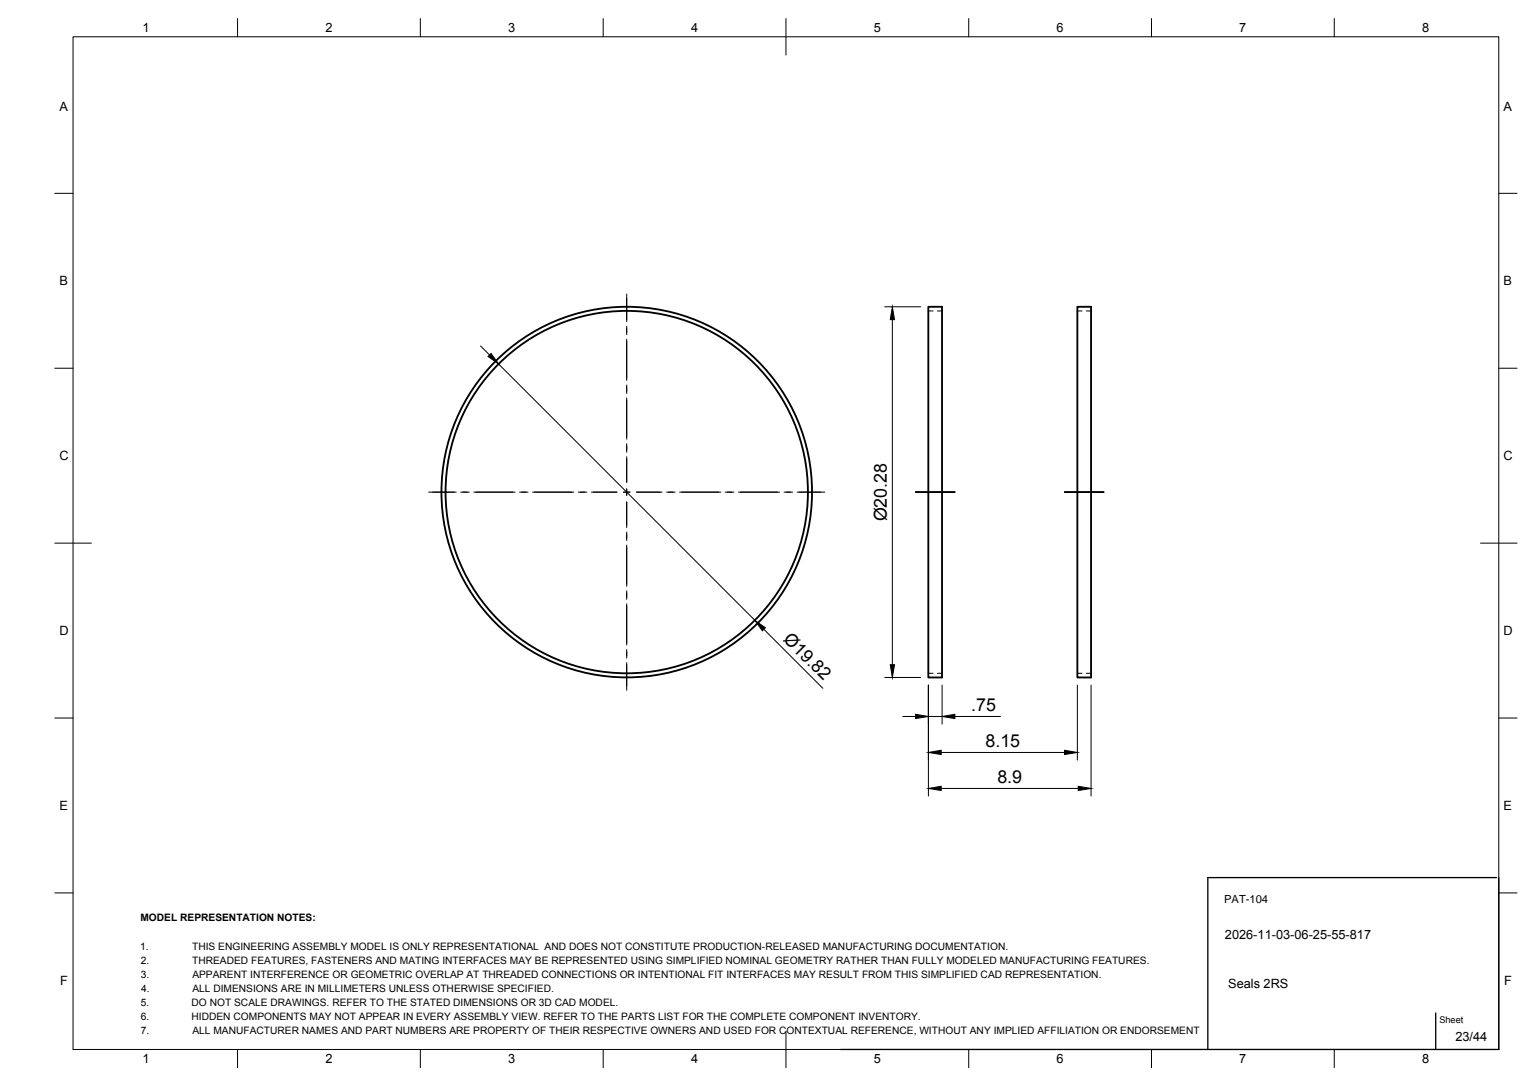
ISO-10303-21;
HEADER;
/* Generated by software containing ST-Developer
 * from STEP Tools, Inc. (www.steptools.com) 
 */

FILE_DESCRIPTION(
/* description */ ('Timing belt drive module 2 mm Pitch Timing 20T-40T'),

/* implementation_level */ '2;1');

FILE_NAME(
/* name */ 'Seals 2RS.step',
/* time_stamp */ '2026-10-28T03:25:12-07:00',
/* author */ (''),
/* organization */ (''),
/* preprocessor_version */ 'ST-DEVELOPER v20.2',
/* originating_system */ 'Autodesk Translation Framework v15.17.0.0',
/* authorisation */ '');

FILE_SCHEMA (('AUTOMOTIVE_DESIGN { 1 0 10303 214 3 1 1 }'));
ENDSEC;

DATA;
#10=MECHANICAL_DESIGN_GEOMETRIC_PRESENTATION_REPRESENTATION('',(#551,#552),#17830);
#458=SHAPE_REPRESENTATION_RELATIONSHIP('SRR','None',#18029,#501);
#501=ADVANCED_BREP_SHAPE_REPRESENTATION('',(#609,#610),#17804);
#551=STYLED_ITEM('',(#18317),#609);
#552=STYLED_ITEM('',(#18317),#610);
#609=MANIFOLD_SOLID_BREP('Body1',#9008);
#610=MANIFOLD_SOLID_BREP('Body2',#9009);
#714=FACE_BOUND('',#1770,.T.);
#715=FACE_BOUND('',#1773,.T.);
#716=FACE_BOUND('',#1776,.T.);
#717=FACE_BOUND('',#1779,.T.);
#866=PLANE('',#9989);
#867=PLANE('',#9994);
#868=PLANE('',#9997);
#869=PLANE('',#10002);
#1171=FACE_OUTER_BOUND('',#1769,.T.);
#1172=FACE_OUTER_BOUND('',#1771,.T.);
#1173=FACE_OUTER_BOUND('',#1772,.T.);
#1174=FACE_OUTER_BOUND('',#1774,.T.);
#1175=FACE_OUTER_BOUND('',#1775,.T.);
#1176=FACE_OUTER_BOUND('',#1777,.T.);
#1177=FACE_OUTER_BOUND('',#1778,.T.);
#1178=FACE_OUTER_BOUND('',#1780,.T.);
#1769=EDGE_LOOP('',(#6729));
#1770=EDGE_LOOP('',(#6730));
#1771=EDGE_LOOP('',(#6731,#6732,#6733,#6734));
#1772=EDGE_LOOP('',(#6735));
#1773=EDGE_LOOP('',(#6736));
#1774=EDGE_LOOP('',(#6737,#6738,#6739,#6740));
#1775=EDGE_LOOP('',(#6741));
#1776=EDGE_LOOP('',(#6742));
#1777=EDGE_LOOP('',(#6743,#6744,#6745,#6746));
#1778=EDGE_LOOP('',(#6747));
#1779=EDGE_LOOP('',(#6748));
#1780=EDGE_LOOP('',(#6749,#6750,#6751,#6752));
#2380=CIRCLE('',#9990,1.013815);
#2381=CIRCLE('',#9991,0.991185);
#2382=CIRCLE('',#9993,1.013815);
#2383=CIRCLE('',#9995,0.991185);
#2384=CIRCLE('',#9998,1.013815);
#2385=CIRCLE('',#9999,0.991185);
#2386=CIRCLE('',#10001,1.013815);
#2387=CIRCLE('',#10003,0.991185);
#3010=LINE('',#15258,#3488);
#3011=LINE('',#15263,#3489);
#3012=LINE('',#15272,#3490);
#3013=LINE('',#15277,#3491);
#3488=VECTOR('',#11985,1.013815);
#3489=VECTOR('',#11992,0.991185);
#3490=VECTOR('',#12003,1.013815);
#3491=VECTOR('',#12010,0.991185);
#4074=VERTEX_POINT('',#15251);
#4075=VERTEX_POINT('',#15253);
#4076=VERTEX_POINT('',#15256);
#4077=VERTEX_POINT('',#15260);
#4078=VERTEX_POINT('',#15265);
#4079=VERTEX_POINT('',#15267);
#4080=VERTEX_POINT('',#15270);
#4081=VERTEX_POINT('',#15274);
#5047=EDGE_CURVE('',#4074,#4074,#2380,.T.);
#5048=EDGE_CURVE('',#4075,#4075,#2381,.T.);
#5049=EDGE_CURVE('',#4076,#4076,#2382,.T.);
#5050=EDGE_CURVE('',#4076,#4074,#3010,.T.);
#5051=EDGE_CURVE('',#4077,#4077,#2383,.T.);
#5052=EDGE_CURVE('',#4077,#4075,#3011,.T.);
#5053=EDGE_CURVE('',#4078,#4078,#2384,.T.);
#5054=EDGE_CURVE('',#4079,#4079,#2385,.T.);
#5055=EDGE_CURVE('',#4080,#4080,#2386,.T.);
#5056=EDGE_CURVE('',#4080,#4078,#3012,.T.);
#5057=EDGE_CURVE('',#4081,#4081,#2387,.T.);
#5058=EDGE_CURVE('',#4081,#4079,#3013,.T.);
#6729=ORIENTED_EDGE('',*,*,#5047,.F.);
#6730=ORIENTED_EDGE('',*,*,#5048,.T.);
#6731=ORIENTED_EDGE('',*,*,#5049,.F.);
#6732=ORIENTED_EDGE('',*,*,#5050,.T.);
#6733=ORIENTED_EDGE('',*,*,#5047,.T.);
#6734=ORIENTED_EDGE('',*,*,#5050,.F.);
#6735=ORIENTED_EDGE('',*,*,#5049,.T.);
#6736=ORIENTED_EDGE('',*,*,#5051,.F.);
#6737=ORIENTED_EDGE('',*,*,#5051,.T.);
#6738=ORIENTED_EDGE('',*,*,#5052,.T.);
#6739=ORIENTED_EDGE('',*,*,#5048,.F.);
#6740=ORIENTED_EDGE('',*,*,#5052,.F.);
#6741=ORIENTED_EDGE('',*,*,#5053,.F.);
#6742=ORIENTED_EDGE('',*,*,#5054,.T.);
#6743=ORIENTED_EDGE('',*,*,#5055,.F.);
#6744=ORIENTED_EDGE('',*,*,#5056,.T.);
#6745=ORIENTED_EDGE('',*,*,#5053,.T.);
#6746=ORIENTED_EDGE('',*,*,#5056,.F.);
#6747=ORIENTED_EDGE('',*,*,#5055,.T.);
#6748=ORIENTED_EDGE('',*,*,#5057,.F.);
#6749=ORIENTED_EDGE('',*,*,#5057,.T.);
#6750=ORIENTED_EDGE('',*,*,#5058,.T.);
#6751=ORIENTED_EDGE('',*,*,#5054,.F.);
#6752=ORIENTED_EDGE('',*,*,#5058,.F.);
#8275=CYLINDRICAL_SURFACE('',#9992,1.013815);
#8276=CYLINDRICAL_SURFACE('',#9996,0.991185);
#8277=CYLINDRICAL_SURFACE('',#10000,1.013815);
#8278=CYLINDRICAL_SURFACE('',#10004,0.991185);
#8669=ADVANCED_FACE('',(#1171,#714),#866,.T.);
#8670=ADVANCED_FACE('',(#1172),#8275,.T.);
#8671=ADVANCED_FACE('',(#1173,#715),#867,.T.);
#8672=ADVANCED_FACE('',(#1174),#8276,.F.);
#8673=ADVANCED_FACE('',(#1175,#716),#868,.T.);
#8674=ADVANCED_FACE('',(#1176),#8277,.T.);
#8675=ADVANCED_FACE('',(#1177,#717),#869,.T.);
#8676=ADVANCED_FACE('',(#1178),#8278,.F.);
#9008=CLOSED_SHELL('',(#8669,#8670,#8671,#8672));
#9009=CLOSED_SHELL('',(#8673,#8674,#8675,#8676));
#9988=AXIS2_PLACEMENT_3D('',#15249,#11973,#11974);
#9989=AXIS2_PLACEMENT_3D('',#15250,#11975,#11976);
#9990=AXIS2_PLACEMENT_3D('',#15252,#11977,#11978);
#9991=AXIS2_PLACEMENT_3D('',#15254,#11979,#11980);
#9992=AXIS2_PLACEMENT_3D('',#15255,#11981,#11982);
#9993=AXIS2_PLACEMENT_3D('',#15257,#11983,#11984);
#9994=AXIS2_PLACEMENT_3D('',#15259,#11986,#11987);
#9995=AXIS2_PLACEMENT_3D('',#15261,#11988,#11989);
#9996=AXIS2_PLACEMENT_3D('',#15262,#11990,#11991);
#9997=AXIS2_PLACEMENT_3D('',#15264,#11993,#11994);
#9998=AXIS2_PLACEMENT_3D('',#15266,#11995,#11996);
#9999=AXIS2_PLACEMENT_3D('',#15268,#11997,#11998);
#10000=AXIS2_PLACEMENT_3D('',#15269,#11999,#12000);
#10001=AXIS2_PLACEMENT_3D('',#15271,#12001,#12002);
#10002=AXIS2_PLACEMENT_3D('',#15273,#12004,#12005);
#10003=AXIS2_PLACEMENT_3D('',#15275,#12006,#12007);
#10004=AXIS2_PLACEMENT_3D('',#15276,#12008,#12009);
#11973=DIRECTION('axis',(0.,0.,1.));
#11974=DIRECTION('refdir',(1.,0.,0.));
#11975=DIRECTION('center_axis',(0.,1.,0.));
#11976=DIRECTION('ref_axis',(0.,0.,1.));
#11977=DIRECTION('center_axis',(0.,-1.,0.));
#11978=DIRECTION('ref_axis',(1.,0.,0.));
#11979=DIRECTION('center_axis',(0.,-1.,0.));
#11980=DIRECTION('ref_axis',(1.,0.,0.));
#11981=DIRECTION('center_axis',(0.,-1.,0.));
#11982=DIRECTION('ref_axis',(1.,0.,0.));
#11983=DIRECTION('center_axis',(0.,-1.,0.));
#11984=DIRECTION('ref_axis',(1.,0.,0.));
#11985=DIRECTION('',(0.,1.,0.));
#11986=DIRECTION('center_axis',(0.,-1.,0.));
#11987=DIRECTION('ref_axis',(0.,0.,-1.));
#11988=DIRECTION('center_axis',(0.,-1.,0.));
#11989=DIRECTION('ref_axis',(1.,0.,0.));
#11990=DIRECTION('center_axis',(0.,-1.,0.));
#11991=DIRECTION('ref_axis',(1.,0.,0.));
#11992=DIRECTION('',(0.,1.,0.));
#11993=DIRECTION('center_axis',(0.,1.,0.));
#11994=DIRECTION('ref_axis',(0.,0.,1.));
#11995=DIRECTION('center_axis',(0.,-1.,0.));
#11996=DIRECTION('ref_axis',(1.,0.,0.));
#11997=DIRECTION('center_axis',(0.,-1.,0.));
#11998=DIRECTION('ref_axis',(1.,0.,0.));
#11999=DIRECTION('center_axis',(0.,-1.,0.));
#12000=DIRECTION('ref_axis',(1.,0.,0.));
#12001=DIRECTION('center_axis',(0.,-1.,0.));
#12002=DIRECTION('ref_axis',(1.,0.,0.));
#12003=DIRECTION('',(0.,1.,0.));
#12004=DIRECTION('center_axis',(0.,-1.,0.));
#12005=DIRECTION('ref_axis',(0.,0.,-1.));
#12006=DIRECTION('center_axis',(0.,-1.,0.));
#12007=DIRECTION('ref_axis',(1.,0.,0.));
#12008=DIRECTION('center_axis',(0.,-1.,0.));
#12009=DIRECTION('ref_axis',(1.,0.,0.));
#12010=DIRECTION('',(0.,1.,0.));
#15249=CARTESIAN_POINT('',(0.,0.,0.));
#15250=CARTESIAN_POINT('Origin',(1.013815,0.445,0.));
#15251=CARTESIAN_POINT('',(-1.013815,0.445,-1.24156529467757E-16));
#15252=CARTESIAN_POINT('Origin',(0.,0.445,0.));
#15253=CARTESIAN_POINT('',(-0.991185,0.445,-1.21385153761287E-16));
#15254=CARTESIAN_POINT('Origin',(0.,0.445,0.));
#15255=CARTESIAN_POINT('Origin',(0.,0.4075,0.));
#15256=CARTESIAN_POINT('',(-1.013815,0.37,-1.24156529467757E-16));
#15257=CARTESIAN_POINT('Origin',(0.,0.37,0.));
#15258=CARTESIAN_POINT('',(-1.013815,0.4075,-1.24156529467757E-16));
#15259=CARTESIAN_POINT('Origin',(0.991185,0.37,0.));
#15260=CARTESIAN_POINT('',(-0.991185,0.37,-1.21385153761287E-16));
#15261=CARTESIAN_POINT('Origin',(0.,0.37,0.));
#15262=CARTESIAN_POINT('Origin',(0.,0.4075,0.));
#15263=CARTESIAN_POINT('',(-0.991185,0.4075,-1.21385153761287E-16));
#15264=CARTESIAN_POINT('Origin',(1.013815,-0.37,0.));
#15265=CARTESIAN_POINT('',(-1.013815,-0.37,-1.24156529467757E-16));
#15266=CARTESIAN_POINT('Origin',(0.,-0.37,0.));
#15267=CARTESIAN_POINT('',(-0.991185,-0.37,-1.21385153761287E-16));
#15268=CARTESIAN_POINT('Origin',(0.,-0.37,0.));
#15269=CARTESIAN_POINT('Origin',(0.,-0.4075,0.));
#15270=CARTESIAN_POINT('',(-1.013815,-0.445,-1.24156529467757E-16));
#15271=CARTESIAN_POINT('Origin',(0.,-0.445,0.));
#15272=CARTESIAN_POINT('',(-1.013815,-0.4075,-1.24156529467757E-16));
#15273=CARTESIAN_POINT('Origin',(0.991185,-0.445,0.));
#15274=CARTESIAN_POINT('',(-0.991185,-0.445,-1.21385153761287E-16));
#15275=CARTESIAN_POINT('Origin',(0.,-0.445,0.));
#15276=CARTESIAN_POINT('Origin',(0.,-0.4075,0.));
#15277=CARTESIAN_POINT('',(-0.991185,-0.4075,-1.21385153761287E-16));
#17754=UNCERTAINTY_MEASURE_WITH_UNIT(LENGTH_MEASURE(0.001),#17831,
'DISTANCE_ACCURACY_VALUE',
'Maximum model space distance between geometric entities at asserted c
onnectivities');
#17780=UNCERTAINTY_MEASURE_WITH_UNIT(LENGTH_MEASURE(0.001),#17831,
'DISTANCE_ACCURACY_VALUE',
'Maximum model space distance between geometric entities at asserted c
onnectivities');
#17804=(
GEOMETRIC_REPRESENTATION_CONTEXT(3)
GLOBAL_UNCERTAINTY_ASSIGNED_CONTEXT((#17754))
GLOBAL_UNIT_ASSIGNED_CONTEXT((#17831,#17833,#17834))
REPRESENTATION_CONTEXT('','3D')
);
#17830=(
GEOMETRIC_REPRESENTATION_CONTEXT(3)
GLOBAL_UNCERTAINTY_ASSIGNED_CONTEXT((#17780))
GLOBAL_UNIT_ASSIGNED_CONTEXT((#17831,#17833,#17834))
REPRESENTATION_CONTEXT('','3D')
);
#17831=(
LENGTH_UNIT()
NAMED_UNIT(*)
SI_UNIT(.CENTI.,.METRE.)
);
#17833=(
NAMED_UNIT(*)
PLANE_ANGLE_UNIT()
SI_UNIT($,.RADIAN.)
);
#17834=(
NAMED_UNIT(*)
SI_UNIT($,.STERADIAN.)
SOLID_ANGLE_UNIT()
);
#17858=SHAPE_DEFINITION_REPRESENTATION(#17907,#18029);
#17907=PRODUCT_DEFINITION_SHAPE('',$,#18079);
#18029=SHAPE_REPRESENTATION('',(#9988),#17804);
#18055=PRODUCT_DEFINITION_CONTEXT('part definition',#18204,'design');
#18079=PRODUCT_DEFINITION('Seals 2RS','Seals 2RS',#18128,#18055);
#18128=PRODUCT_DEFINITION_FORMATION('',$,#18229);
#18204=APPLICATION_CONTEXT(
'Core Data for Automotive Mechanical Design Process');
#18205=PRODUCT_CONTEXT('part definition',#18204,'mechanical');
#18229=PRODUCT('Seals 2RS','Seals 2RS','Seals 2RS',(#18205));
#18311=COLOUR_RGB('Grey',0.48,0.52,0.57);
#18312=FILL_AREA_STYLE_COLOUR('',#18311);
#18313=FILL_AREA_STYLE('',(#18312));
#18314=SURFACE_STYLE_FILL_AREA(#18313);
#18315=SURFACE_SIDE_STYLE('',(#18314));
#18316=SURFACE_STYLE_USAGE(.BOTH.,#18315);
#18317=PRESENTATION_STYLE_ASSIGNMENT((#18316));
ENDSEC;
END-ISO-10303-21;
